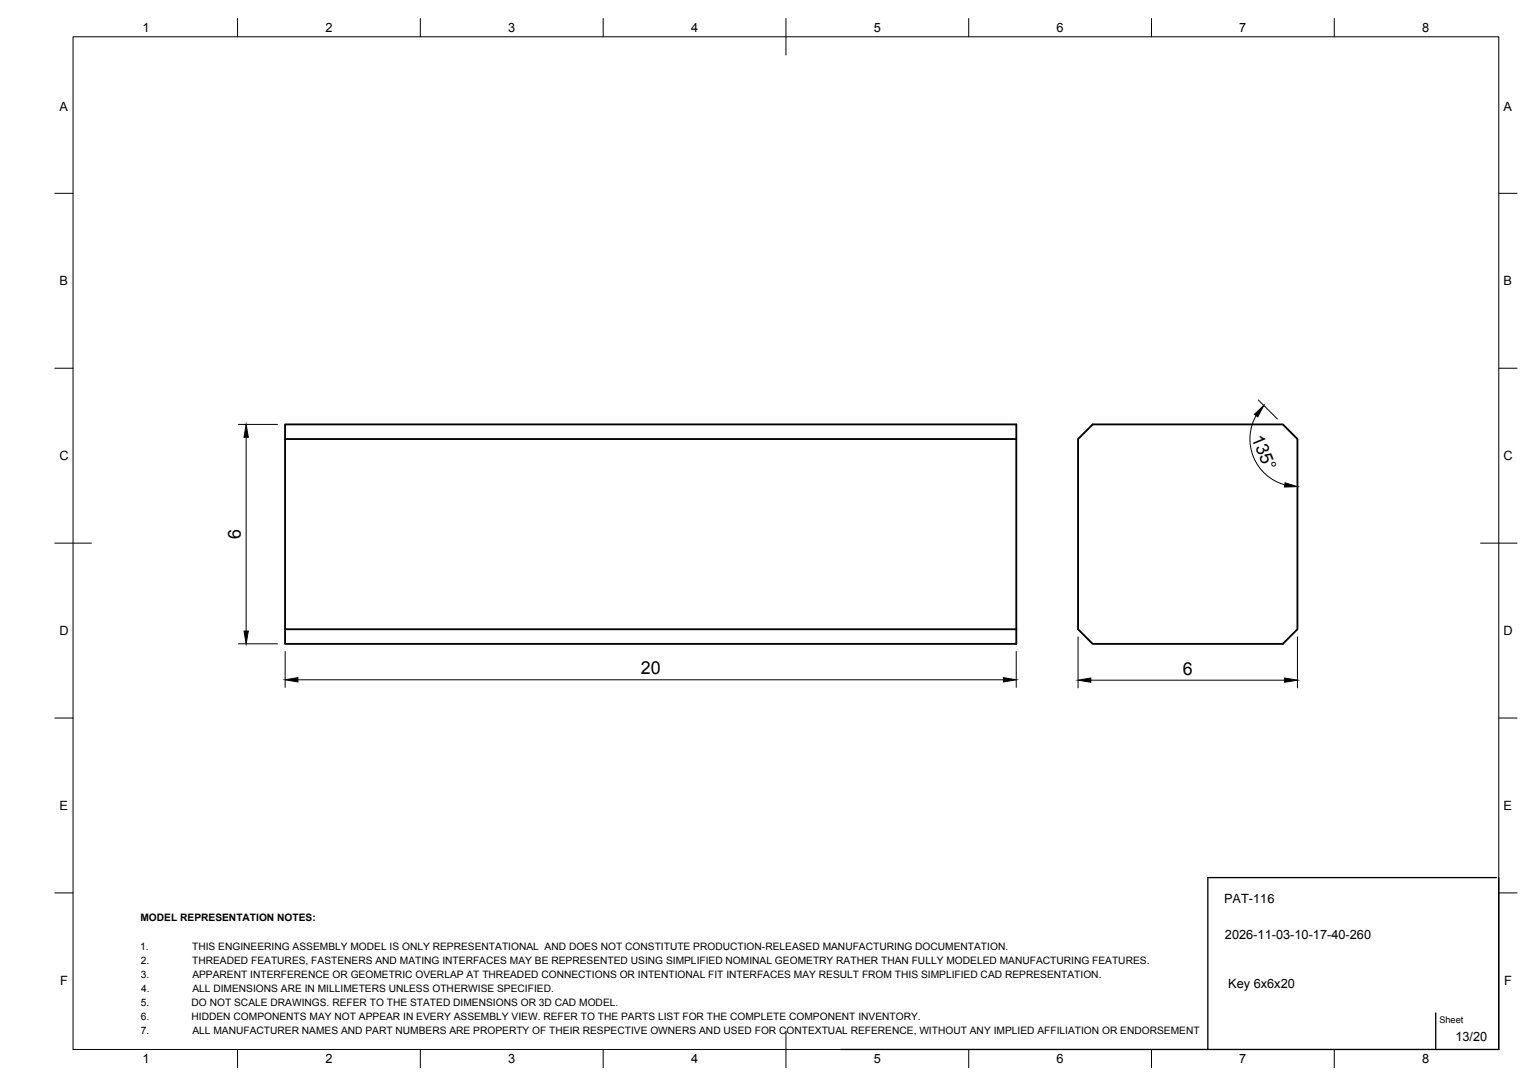
ISO-10303-21;
HEADER;
/* Generated by software containing ST-Developer
 * from STEP Tools, Inc. (www.steptools.com) 
 */

FILE_DESCRIPTION(
/* description */ ('V-block with clamp strap'),
/* implementation_level */ '2;1');

FILE_NAME(
/* name */ 'Key 6x6x20.step',
/* time_stamp */ '2026-10-27T10:50:53-07:00',
/* author */ (''),
/* organization */ (''),
/* preprocessor_version */ 'ST-DEVELOPER v20.2',
/* originating_system */ 'Autodesk Translation Framework v15.17.0.0',
/* authorisation */ '');

FILE_SCHEMA (('AUTOMOTIVE_DESIGN { 1 0 10303 214 3 1 1 }'));
ENDSEC;

DATA;
#10=MECHANICAL_DESIGN_GEOMETRIC_PRESENTATION_REPRESENTATION('',(#274),#7344);
#232=SHAPE_REPRESENTATION_RELATIONSHIP('SRR','None',#7450,#253);
#253=ADVANCED_BREP_SHAPE_REPRESENTATION('',(#295),#7329);
#274=STYLED_ITEM('',(#7631),#295);
#295=MANIFOLD_SOLID_BREP('Body1',#4156);
#683=FACE_OUTER_BOUND('',#973,.T.);
#684=FACE_OUTER_BOUND('',#974,.T.);
#685=FACE_OUTER_BOUND('',#975,.T.);
#686=FACE_OUTER_BOUND('',#976,.T.);
#687=FACE_OUTER_BOUND('',#977,.T.);
#688=FACE_OUTER_BOUND('',#978,.T.);
#689=FACE_OUTER_BOUND('',#979,.T.);
#690=FACE_OUTER_BOUND('',#980,.T.);
#691=FACE_OUTER_BOUND('',#981,.T.);
#692=FACE_OUTER_BOUND('',#982,.T.);
#973=EDGE_LOOP('',(#3278,#3279,#3280,#3281,#3282,#3283,#3284,#3285));
#974=EDGE_LOOP('',(#3286,#3287,#3288,#3289));
#975=EDGE_LOOP('',(#3290,#3291,#3292,#3293));
#976=EDGE_LOOP('',(#3294,#3295,#3296,#3297));
#977=EDGE_LOOP('',(#3298,#3299,#3300,#3301));
#978=EDGE_LOOP('',(#3302,#3303,#3304,#3305,#3306,#3307,#3308,#3309));
#979=EDGE_LOOP('',(#3310,#3311,#3312,#3313));
#980=EDGE_LOOP('',(#3314,#3315,#3316,#3317));
#981=EDGE_LOOP('',(#3318,#3319,#3320,#3321));
#982=EDGE_LOOP('',(#3322,#3323,#3324,#3325));
#1330=LINE('',#6694,#1695);
#1331=LINE('',#6696,#1696);
#1332=LINE('',#6698,#1697);
#1333=LINE('',#6700,#1698);
#1334=LINE('',#6702,#1699);
#1335=LINE('',#6704,#1700);
#1336=LINE('',#6706,#1701);
#1337=LINE('',#6707,#1702);
#1338=LINE('',#6710,#1703);
#1339=LINE('',#6712,#1704);
#1340=LINE('',#6713,#1705);
#1341=LINE('',#6716,#1706);
#1342=LINE('',#6717,#1707);
#1343=LINE('',#6720,#1708);
#1344=LINE('',#6721,#1709);
#1345=LINE('',#6724,#1710);
#1346=LINE('',#6725,#1711);
#1347=LINE('',#6729,#1712);
#1348=LINE('',#6730,#1713);
#1349=LINE('',#6732,#1714);
#1350=LINE('',#6733,#1715);
#1351=LINE('',#6735,#1716);
#1352=LINE('',#6737,#1717);
#1353=LINE('',#6739,#1718);
#1695=VECTOR('',#5474,1.);
#1696=VECTOR('',#5475,1.);
#1697=VECTOR('',#5476,1.);
#1698=VECTOR('',#5477,1.);
#1699=VECTOR('',#5478,1.);
#1700=VECTOR('',#5479,1.);
#1701=VECTOR('',#5480,1.);
#1702=VECTOR('',#5481,1.);
#1703=VECTOR('',#5484,1.);
#1704=VECTOR('',#5485,1.);
#1705=VECTOR('',#5486,1.);
#1706=VECTOR('',#5489,1.);
#1707=VECTOR('',#5490,1.);
#1708=VECTOR('',#5493,1.);
#1709=VECTOR('',#5494,1.);
#1710=VECTOR('',#5497,1.);
#1711=VECTOR('',#5498,1.);
#1712=VECTOR('',#5501,1.);
#1713=VECTOR('',#5502,1.);
#1714=VECTOR('',#5503,1.);
#1715=VECTOR('',#5504,1.);
#1716=VECTOR('',#5507,1.);
#1717=VECTOR('',#5510,1.);
#1718=VECTOR('',#5513,1.);
#2025=VERTEX_POINT('',#6692);
#2026=VERTEX_POINT('',#6693);
#2027=VERTEX_POINT('',#6695);
#2028=VERTEX_POINT('',#6697);
#2029=VERTEX_POINT('',#6699);
#2030=VERTEX_POINT('',#6701);
#2031=VERTEX_POINT('',#6703);
#2032=VERTEX_POINT('',#6705);
#2033=VERTEX_POINT('',#6709);
#2034=VERTEX_POINT('',#6711);
#2035=VERTEX_POINT('',#6715);
#2036=VERTEX_POINT('',#6719);
#2037=VERTEX_POINT('',#6723);
#2038=VERTEX_POINT('',#6727);
#2039=VERTEX_POINT('',#6728);
#2040=VERTEX_POINT('',#6731);
#2465=EDGE_CURVE('',#2025,#2026,#1330,.T.);
#2466=EDGE_CURVE('',#2027,#2025,#1331,.T.);
#2467=EDGE_CURVE('',#2028,#2027,#1332,.T.);
#2468=EDGE_CURVE('',#2029,#2028,#1333,.T.);
#2469=EDGE_CURVE('',#2030,#2029,#1334,.T.);
#2470=EDGE_CURVE('',#2031,#2030,#1335,.T.);
#2471=EDGE_CURVE('',#2032,#2031,#1336,.T.);
#2472=EDGE_CURVE('',#2026,#2032,#1337,.T.);
#2473=EDGE_CURVE('',#2029,#2033,#1338,.T.);
#2474=EDGE_CURVE('',#2033,#2034,#1339,.T.);
#2475=EDGE_CURVE('',#2034,#2030,#1340,.T.);
#2476=EDGE_CURVE('',#2035,#2028,#1341,.T.);
#2477=EDGE_CURVE('',#2035,#2033,#1342,.T.);
#2478=EDGE_CURVE('',#2027,#2036,#1343,.T.);
#2479=EDGE_CURVE('',#2036,#2035,#1344,.T.);
#2480=EDGE_CURVE('',#2037,#2025,#1345,.T.);
#2481=EDGE_CURVE('',#2037,#2036,#1346,.T.);
#2482=EDGE_CURVE('',#2038,#2039,#1347,.T.);
#2483=EDGE_CURVE('',#2034,#2038,#1348,.T.);
#2484=EDGE_CURVE('',#2040,#2037,#1349,.T.);
#2485=EDGE_CURVE('',#2039,#2040,#1350,.T.);
#2486=EDGE_CURVE('',#2031,#2038,#1351,.T.);
#2487=EDGE_CURVE('',#2026,#2040,#1352,.T.);
#2488=EDGE_CURVE('',#2039,#2032,#1353,.T.);
#3278=ORIENTED_EDGE('',*,*,#2465,.F.);
#3279=ORIENTED_EDGE('',*,*,#2466,.F.);
#3280=ORIENTED_EDGE('',*,*,#2467,.F.);
#3281=ORIENTED_EDGE('',*,*,#2468,.F.);
#3282=ORIENTED_EDGE('',*,*,#2469,.F.);
#3283=ORIENTED_EDGE('',*,*,#2470,.F.);
#3284=ORIENTED_EDGE('',*,*,#2471,.F.);
#3285=ORIENTED_EDGE('',*,*,#2472,.F.);
#3286=ORIENTED_EDGE('',*,*,#2469,.T.);
#3287=ORIENTED_EDGE('',*,*,#2473,.T.);
#3288=ORIENTED_EDGE('',*,*,#2474,.T.);
#3289=ORIENTED_EDGE('',*,*,#2475,.T.);
#3290=ORIENTED_EDGE('',*,*,#2468,.T.);
#3291=ORIENTED_EDGE('',*,*,#2476,.F.);
#3292=ORIENTED_EDGE('',*,*,#2477,.T.);
#3293=ORIENTED_EDGE('',*,*,#2473,.F.);
#3294=ORIENTED_EDGE('',*,*,#2467,.T.);
#3295=ORIENTED_EDGE('',*,*,#2478,.T.);
#3296=ORIENTED_EDGE('',*,*,#2479,.T.);
#3297=ORIENTED_EDGE('',*,*,#2476,.T.);
#3298=ORIENTED_EDGE('',*,*,#2466,.T.);
#3299=ORIENTED_EDGE('',*,*,#2480,.F.);
#3300=ORIENTED_EDGE('',*,*,#2481,.T.);
#3301=ORIENTED_EDGE('',*,*,#2478,.F.);
#3302=ORIENTED_EDGE('',*,*,#2482,.F.);
#3303=ORIENTED_EDGE('',*,*,#2483,.F.);
#3304=ORIENTED_EDGE('',*,*,#2474,.F.);
#3305=ORIENTED_EDGE('',*,*,#2477,.F.);
#3306=ORIENTED_EDGE('',*,*,#2479,.F.);
#3307=ORIENTED_EDGE('',*,*,#2481,.F.);
#3308=ORIENTED_EDGE('',*,*,#2484,.F.);
#3309=ORIENTED_EDGE('',*,*,#2485,.F.);
#3310=ORIENTED_EDGE('',*,*,#2470,.T.);
#3311=ORIENTED_EDGE('',*,*,#2475,.F.);
#3312=ORIENTED_EDGE('',*,*,#2483,.T.);
#3313=ORIENTED_EDGE('',*,*,#2486,.F.);
#3314=ORIENTED_EDGE('',*,*,#2465,.T.);
#3315=ORIENTED_EDGE('',*,*,#2487,.T.);
#3316=ORIENTED_EDGE('',*,*,#2484,.T.);
#3317=ORIENTED_EDGE('',*,*,#2480,.T.);
#3318=ORIENTED_EDGE('',*,*,#2471,.T.);
#3319=ORIENTED_EDGE('',*,*,#2486,.T.);
#3320=ORIENTED_EDGE('',*,*,#2482,.T.);
#3321=ORIENTED_EDGE('',*,*,#2488,.T.);
#3322=ORIENTED_EDGE('',*,*,#2472,.T.);
#3323=ORIENTED_EDGE('',*,*,#2488,.F.);
#3324=ORIENTED_EDGE('',*,*,#2485,.T.);
#3325=ORIENTED_EDGE('',*,*,#2487,.F.);
#3826=PLANE('',#4610);
#3827=PLANE('',#4611);
#3828=PLANE('',#4612);
#3829=PLANE('',#4613);
#3830=PLANE('',#4614);
#3831=PLANE('',#4615);
#3832=PLANE('',#4616);
#3833=PLANE('',#4617);
#3834=PLANE('',#4618);
#3835=PLANE('',#4619);
#4029=ADVANCED_FACE('',(#683),#3826,.F.);
#4030=ADVANCED_FACE('',(#684),#3827,.T.);
#4031=ADVANCED_FACE('',(#685),#3828,.T.);
#4032=ADVANCED_FACE('',(#686),#3829,.T.);
#4033=ADVANCED_FACE('',(#687),#3830,.T.);
#4034=ADVANCED_FACE('',(#688),#3831,.T.);
#4035=ADVANCED_FACE('',(#689),#3832,.F.);
#4036=ADVANCED_FACE('',(#690),#3833,.T.);
#4037=ADVANCED_FACE('',(#691),#3834,.T.);
#4038=ADVANCED_FACE('',(#692),#3835,.T.);
#4156=CLOSED_SHELL('',(#4029,#4030,#4031,#4032,#4033,#4034,#4035,#4036,
#4037,#4038));
#4609=AXIS2_PLACEMENT_3D('',#6690,#5470,#5471);
#4610=AXIS2_PLACEMENT_3D('',#6691,#5472,#5473);
#4611=AXIS2_PLACEMENT_3D('',#6708,#5482,#5483);
#4612=AXIS2_PLACEMENT_3D('',#6714,#5487,#5488);
#4613=AXIS2_PLACEMENT_3D('',#6718,#5491,#5492);
#4614=AXIS2_PLACEMENT_3D('',#6722,#5495,#5496);
#4615=AXIS2_PLACEMENT_3D('',#6726,#5499,#5500);
#4616=AXIS2_PLACEMENT_3D('',#6734,#5505,#5506);
#4617=AXIS2_PLACEMENT_3D('',#6736,#5508,#5509);
#4618=AXIS2_PLACEMENT_3D('',#6738,#5511,#5512);
#4619=AXIS2_PLACEMENT_3D('',#6740,#5514,#5515);
#5470=DIRECTION('axis',(0.,0.,1.));
#5471=DIRECTION('refdir',(1.,0.,0.));
#5472=DIRECTION('center_axis',(1.,0.,0.));
#5473=DIRECTION('ref_axis',(0.,0.,-1.));
#5474=DIRECTION('',(0.,-0.707106781186547,-0.707106781186548));
#5475=DIRECTION('',(0.,-1.,0.));
#5476=DIRECTION('',(0.,-0.707106781186547,0.707106781186548));
#5477=DIRECTION('',(0.,0.,1.));
#5478=DIRECTION('',(0.,0.707106781186547,0.707106781186548));
#5479=DIRECTION('',(0.,1.,0.));
#5480=DIRECTION('',(0.,0.707106781186547,-0.707106781186548));
#5481=DIRECTION('',(0.,0.,-1.));
#5482=DIRECTION('center_axis',(0.,0.707106781186548,-0.707106781186547));
#5483=DIRECTION('ref_axis',(-1.,0.,0.));
#5484=DIRECTION('',(1.,0.,0.));
#5485=DIRECTION('',(0.,-0.707106781186547,-0.707106781186548));
#5486=DIRECTION('',(-1.,0.,0.));
#5487=DIRECTION('center_axis',(0.,1.,0.));
#5488=DIRECTION('ref_axis',(-1.,0.,0.));
#5489=DIRECTION('',(-1.,0.,0.));
#5490=DIRECTION('',(0.,0.,-1.));
#5491=DIRECTION('center_axis',(0.,0.707106781186548,0.707106781186547));
#5492=DIRECTION('ref_axis',(1.,0.,0.));
#5493=DIRECTION('',(1.,0.,0.));
#5494=DIRECTION('',(0.,0.707106781186547,-0.707106781186548));
#5495=DIRECTION('center_axis',(0.,0.,1.));
#5496=DIRECTION('ref_axis',(1.,0.,0.));
#5497=DIRECTION('',(-1.,0.,0.));
#5498=DIRECTION('',(0.,1.,0.));
#5499=DIRECTION('center_axis',(1.,0.,0.));
#5500=DIRECTION('ref_axis',(0.,0.,-1.));
#5501=DIRECTION('',(0.,-0.707106781186547,0.707106781186548));
#5502=DIRECTION('',(0.,-1.,0.));
#5503=DIRECTION('',(0.,0.707106781186547,0.707106781186548));
#5504=DIRECTION('',(0.,0.,1.));
#5505=DIRECTION('center_axis',(0.,0.,1.));
#5506=DIRECTION('ref_axis',(1.,0.,0.));
#5507=DIRECTION('',(1.,0.,0.));
#5508=DIRECTION('center_axis',(0.,-0.707106781186548,0.707106781186547));
#5509=DIRECTION('ref_axis',(1.,0.,0.));
#5510=DIRECTION('',(1.,0.,0.));
#5511=DIRECTION('center_axis',(0.,-0.707106781186548,-0.707106781186547));
#5512=DIRECTION('ref_axis',(-1.,0.,0.));
#5513=DIRECTION('',(-1.,0.,0.));
#5514=DIRECTION('center_axis',(0.,-1.,0.));
#5515=DIRECTION('ref_axis',(1.,0.,0.));
#6690=CARTESIAN_POINT('',(0.,0.,0.));
#6691=CARTESIAN_POINT('Origin',(-1.,0.,0.35));
#6692=CARTESIAN_POINT('',(-1.,-0.26,0.6));
#6693=CARTESIAN_POINT('',(-1.,-0.3,0.56));
#6694=CARTESIAN_POINT('',(-1.,-0.2675,0.5925));
#6695=CARTESIAN_POINT('',(-1.,0.26,0.6));
#6696=CARTESIAN_POINT('',(-1.,0.,0.6));
#6697=CARTESIAN_POINT('',(-1.,0.3,0.56));
#6698=CARTESIAN_POINT('',(-1.,0.2675,0.5925));
#6699=CARTESIAN_POINT('',(-1.,0.3,0.04));
#6700=CARTESIAN_POINT('',(-1.,0.3,0.175));
#6701=CARTESIAN_POINT('',(-1.,0.26,0.));
#6702=CARTESIAN_POINT('',(-1.,0.2925,0.0325));
#6703=CARTESIAN_POINT('',(-1.,-0.26,0.));
#6704=CARTESIAN_POINT('',(-1.,0.,0.));
#6705=CARTESIAN_POINT('',(-1.,-0.3,0.04));
#6706=CARTESIAN_POINT('',(-1.,-0.2925,0.0325));
#6707=CARTESIAN_POINT('',(-1.,-0.3,0.175));
#6708=CARTESIAN_POINT('Origin',(0.75,0.28,0.02));
#6709=CARTESIAN_POINT('',(1.,0.3,0.04));
#6710=CARTESIAN_POINT('',(0.75,0.3,0.04));
#6711=CARTESIAN_POINT('',(1.,0.26,0.));
#6712=CARTESIAN_POINT('',(1.,0.2925,0.0325));
#6713=CARTESIAN_POINT('',(0.75,0.26,0.));
#6714=CARTESIAN_POINT('Origin',(1.5,0.3,0.));
#6715=CARTESIAN_POINT('',(1.,0.3,0.56));
#6716=CARTESIAN_POINT('',(0.75,0.3,0.56));
#6717=CARTESIAN_POINT('',(1.,0.3,0.175));
#6718=CARTESIAN_POINT('Origin',(0.75,0.28,0.58));
#6719=CARTESIAN_POINT('',(1.,0.26,0.6));
#6720=CARTESIAN_POINT('',(0.75,0.26,0.6));
#6721=CARTESIAN_POINT('',(1.,0.2675,0.5925));
#6722=CARTESIAN_POINT('Origin',(0.,0.,0.6));
#6723=CARTESIAN_POINT('',(1.,-0.26,0.6));
#6724=CARTESIAN_POINT('',(-0.75,-0.26,0.6));
#6725=CARTESIAN_POINT('',(1.,0.,0.6));
#6726=CARTESIAN_POINT('Origin',(1.,0.,0.35));
#6727=CARTESIAN_POINT('',(1.,-0.26,0.));
#6728=CARTESIAN_POINT('',(1.,-0.3,0.04));
#6729=CARTESIAN_POINT('',(1.,-0.2925,0.0325));
#6730=CARTESIAN_POINT('',(1.,0.,0.));
#6731=CARTESIAN_POINT('',(1.,-0.3,0.56));
#6732=CARTESIAN_POINT('',(1.,-0.2675,0.5925));
#6733=CARTESIAN_POINT('',(1.,-0.3,0.175));
#6734=CARTESIAN_POINT('Origin',(0.,0.,0.));
#6735=CARTESIAN_POINT('',(-0.75,-0.26,0.));
#6736=CARTESIAN_POINT('Origin',(-0.75,-0.28,0.58));
#6737=CARTESIAN_POINT('',(-0.75,-0.3,0.56));
#6738=CARTESIAN_POINT('Origin',(-0.75,-0.28,0.02));
#6739=CARTESIAN_POINT('',(-0.75,-0.3,0.04));
#6740=CARTESIAN_POINT('Origin',(-1.5,-0.3,0.));
#7303=UNCERTAINTY_MEASURE_WITH_UNIT(LENGTH_MEASURE(0.001),#7345,
'DISTANCE_ACCURACY_VALUE',
'Maximum model space distance between geometric entities at asserted c
onnectivities');
#7318=UNCERTAINTY_MEASURE_WITH_UNIT(LENGTH_MEASURE(0.001),#7345,
'DISTANCE_ACCURACY_VALUE',
'Maximum model space distance between geometric entities at asserted c
onnectivities');
#7329=(
GEOMETRIC_REPRESENTATION_CONTEXT(3)
GLOBAL_UNCERTAINTY_ASSIGNED_CONTEXT((#7303))
GLOBAL_UNIT_ASSIGNED_CONTEXT((#7345,#7347,#7348))
REPRESENTATION_CONTEXT('','3D')
);
#7344=(
GEOMETRIC_REPRESENTATION_CONTEXT(3)
GLOBAL_UNCERTAINTY_ASSIGNED_CONTEXT((#7318))
GLOBAL_UNIT_ASSIGNED_CONTEXT((#7345,#7347,#7348))
REPRESENTATION_CONTEXT('','3D')
);
#7345=(
LENGTH_UNIT()
NAMED_UNIT(*)
SI_UNIT(.CENTI.,.METRE.)
);
#7347=(
NAMED_UNIT(*)
PLANE_ANGLE_UNIT()
SI_UNIT($,.RADIAN.)
);
#7348=(
NAMED_UNIT(*)
SI_UNIT($,.STERADIAN.)
SOLID_ANGLE_UNIT()
);
#7359=SHAPE_DEFINITION_REPRESENTATION(#7384,#7450);
#7384=PRODUCT_DEFINITION_SHAPE('',$,#7476);
#7450=SHAPE_REPRESENTATION('',(#4609),#7329);
#7465=PRODUCT_DEFINITION_CONTEXT('part definition',#7542,'design');
#7476=PRODUCT_DEFINITION('Key 6x6x20','Key 6x6x20',#7501,#7465);
#7501=PRODUCT_DEFINITION_FORMATION('',$,#7554);
#7542=APPLICATION_CONTEXT(
'Core Data for Automotive Mechanical Design Process');
#7543=PRODUCT_CONTEXT('part definition',#7542,'mechanical');
#7554=PRODUCT('Key 6x6x20','Key 6x6x20','Key 6x6x20',(#7543));
#7625=COLOUR_RGB('Grey',0.48,0.52,0.57);
#7626=FILL_AREA_STYLE_COLOUR('',#7625);
#7627=FILL_AREA_STYLE('',(#7626));
#7628=SURFACE_STYLE_FILL_AREA(#7627);
#7629=SURFACE_SIDE_STYLE('',(#7628));
#7630=SURFACE_STYLE_USAGE(.BOTH.,#7629);
#7631=PRESENTATION_STYLE_ASSIGNMENT((#7630));
ENDSEC;
END-ISO-10303-21;
